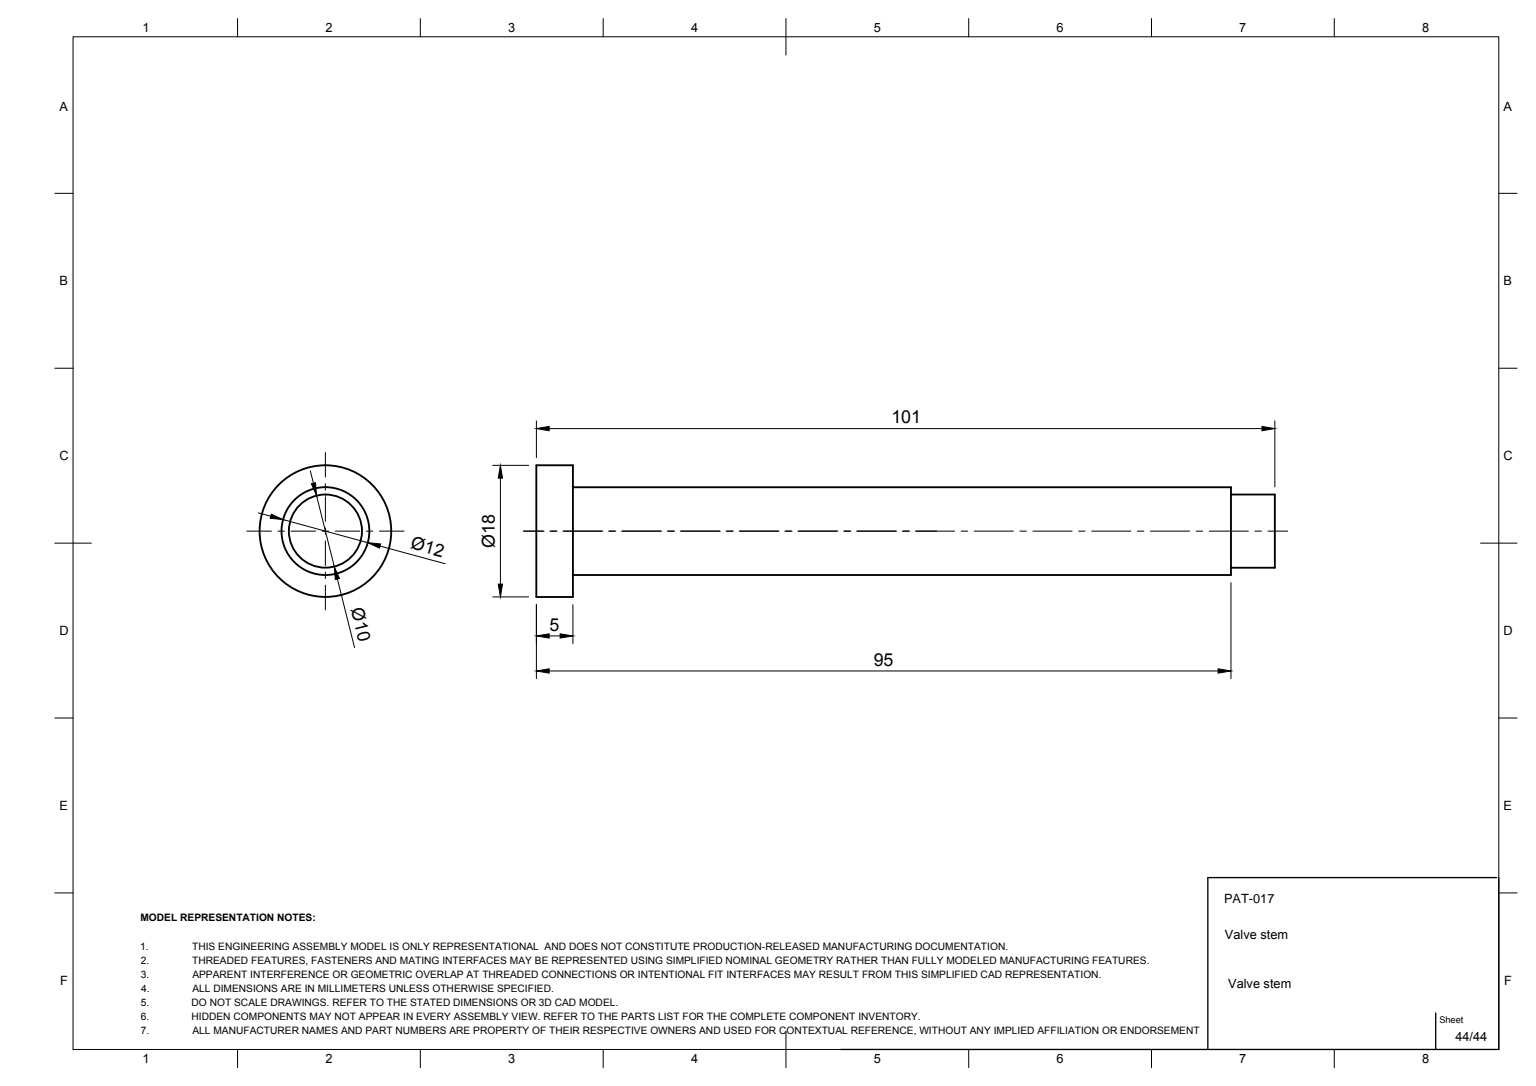
ISO-10303-21;
HEADER;
/* Generated by software containing ST-Developer
 * from STEP Tools, Inc. (www.steptools.com) 
 */

FILE_DESCRIPTION(
/* description */ ('Cam-and-follower valve demonstrator'),
/* implementation_level */ '2;1');

FILE_NAME(
/* name */ 'Valve stem.step',
/* time_stamp */ '2026-10-28T03:25:17-07:00',
/* author */ (''),
/* organization */ (''),
/* preprocessor_version */ 'ST-DEVELOPER v20.2',
/* originating_system */ 'Autodesk Translation Framework v15.17.0.0',
/* authorisation */ '');

FILE_SCHEMA (('AUTOMOTIVE_DESIGN { 1 0 10303 214 3 1 1 }'));
ENDSEC;

DATA;
#10=MECHANICAL_DESIGN_GEOMETRIC_PRESENTATION_REPRESENTATION('',(#453),#12896);
#374=SHAPE_REPRESENTATION_RELATIONSHIP('SRR','None',#13094,#410);
#410=ADVANCED_BREP_SHAPE_REPRESENTATION('',(#493),#12894);
#453=STYLED_ITEM('',(#13344),#493);
#493=MANIFOLD_SOLID_BREP('Body1',#6223);
#655=FACE_BOUND('',#1981,.T.);
#656=FACE_BOUND('',#1988,.T.);
#963=CIRCLE('',#7387,0.9);
#964=CIRCLE('',#7388,0.6);
#965=CIRCLE('',#7390,0.9);
#966=CIRCLE('',#7393,0.5);
#967=CIRCLE('',#7394,0.5);
#968=CIRCLE('',#7397,0.6);
#1090=CYLINDRICAL_SURFACE('',#7389,0.9);
#1091=CYLINDRICAL_SURFACE('',#7392,0.5);
#1092=CYLINDRICAL_SURFACE('',#7396,0.6);
#1452=FACE_OUTER_BOUND('',#1980,.T.);
#1453=FACE_OUTER_BOUND('',#1982,.T.);
#1454=FACE_OUTER_BOUND('',#1983,.T.);
#1455=FACE_OUTER_BOUND('',#1984,.T.);
#1456=FACE_OUTER_BOUND('',#1985,.T.);
#1457=FACE_OUTER_BOUND('',#1986,.T.);
#1458=FACE_OUTER_BOUND('',#1987,.T.);
#1980=EDGE_LOOP('',(#5567));
#1981=EDGE_LOOP('',(#5568));
#1982=EDGE_LOOP('',(#5569,#5570,#5571,#5572));
#1983=EDGE_LOOP('',(#5573));
#1984=EDGE_LOOP('',(#5574,#5575,#5576,#5577));
#1985=EDGE_LOOP('',(#5578));
#1986=EDGE_LOOP('',(#5579,#5580,#5581,#5582));
#1987=EDGE_LOOP('',(#5583));
#1988=EDGE_LOOP('',(#5584));
#2412=LINE('',#12776,#2834);
#2413=LINE('',#12782,#2835);
#2414=LINE('',#12787,#2836);
#2834=VECTOR('',#9369,0.9);
#2835=VECTOR('',#9376,0.5);
#2836=VECTOR('',#9383,0.6);
#3334=VERTEX_POINT('',#12769);
#3335=VERTEX_POINT('',#12771);
#3336=VERTEX_POINT('',#12774);
#3337=VERTEX_POINT('',#12779);
#3338=VERTEX_POINT('',#12781);
#3339=VERTEX_POINT('',#12786);
#4080=EDGE_CURVE('',#3334,#3334,#963,.T.);
#4081=EDGE_CURVE('',#3335,#3335,#964,.T.);
#4082=EDGE_CURVE('',#3336,#3336,#965,.T.);
#4083=EDGE_CURVE('',#3336,#3334,#2412,.T.);
#4084=EDGE_CURVE('',#3337,#3337,#966,.T.);
#4085=EDGE_CURVE('',#3337,#3338,#2413,.T.);
#4086=EDGE_CURVE('',#3338,#3338,#967,.T.);
#4087=EDGE_CURVE('',#3335,#3339,#2414,.T.);
#4088=EDGE_CURVE('',#3339,#3339,#968,.T.);
#5567=ORIENTED_EDGE('',*,*,#4080,.F.);
#5568=ORIENTED_EDGE('',*,*,#4081,.T.);
#5569=ORIENTED_EDGE('',*,*,#4082,.F.);
#5570=ORIENTED_EDGE('',*,*,#4083,.T.);
#5571=ORIENTED_EDGE('',*,*,#4080,.T.);
#5572=ORIENTED_EDGE('',*,*,#4083,.F.);
#5573=ORIENTED_EDGE('',*,*,#4082,.T.);
#5574=ORIENTED_EDGE('',*,*,#4084,.F.);
#5575=ORIENTED_EDGE('',*,*,#4085,.T.);
#5576=ORIENTED_EDGE('',*,*,#4086,.T.);
#5577=ORIENTED_EDGE('',*,*,#4085,.F.);
#5578=ORIENTED_EDGE('',*,*,#4086,.F.);
#5579=ORIENTED_EDGE('',*,*,#4081,.F.);
#5580=ORIENTED_EDGE('',*,*,#4087,.T.);
#5581=ORIENTED_EDGE('',*,*,#4088,.T.);
#5582=ORIENTED_EDGE('',*,*,#4087,.F.);
#5583=ORIENTED_EDGE('',*,*,#4088,.F.);
#5584=ORIENTED_EDGE('',*,*,#4084,.T.);
#5805=PLANE('',#7386);
#5806=PLANE('',#7391);
#5807=PLANE('',#7395);
#5808=PLANE('',#7398);
#6168=ADVANCED_FACE('',(#1452,#655),#5805,.F.);
#6169=ADVANCED_FACE('',(#1453),#1090,.T.);
#6170=ADVANCED_FACE('',(#1454),#5806,.T.);
#6171=ADVANCED_FACE('',(#1455),#1091,.T.);
#6172=ADVANCED_FACE('',(#1456),#5807,.F.);
#6173=ADVANCED_FACE('',(#1457),#1092,.T.);
#6174=ADVANCED_FACE('',(#1458,#656),#5808,.F.);
#6223=CLOSED_SHELL('',(#6168,#6169,#6170,#6171,#6172,#6173,#6174));
#7385=AXIS2_PLACEMENT_3D('',#12767,#9357,#9358);
#7386=AXIS2_PLACEMENT_3D('',#12768,#9359,#9360);
#7387=AXIS2_PLACEMENT_3D('',#12770,#9361,#9362);
#7388=AXIS2_PLACEMENT_3D('',#12772,#9363,#9364);
#7389=AXIS2_PLACEMENT_3D('',#12773,#9365,#9366);
#7390=AXIS2_PLACEMENT_3D('',#12775,#9367,#9368);
#7391=AXIS2_PLACEMENT_3D('',#12777,#9370,#9371);
#7392=AXIS2_PLACEMENT_3D('',#12778,#9372,#9373);
#7393=AXIS2_PLACEMENT_3D('',#12780,#9374,#9375);
#7394=AXIS2_PLACEMENT_3D('',#12783,#9377,#9378);
#7395=AXIS2_PLACEMENT_3D('',#12784,#9379,#9380);
#7396=AXIS2_PLACEMENT_3D('',#12785,#9381,#9382);
#7397=AXIS2_PLACEMENT_3D('',#12788,#9384,#9385);
#7398=AXIS2_PLACEMENT_3D('',#12789,#9386,#9387);
#9357=DIRECTION('axis',(0.,0.,1.));
#9358=DIRECTION('refdir',(1.,0.,0.));
#9359=DIRECTION('center_axis',(0.,0.,1.));
#9360=DIRECTION('ref_axis',(1.,0.,0.));
#9361=DIRECTION('center_axis',(0.,0.,1.));
#9362=DIRECTION('ref_axis',(1.,0.,0.));
#9363=DIRECTION('center_axis',(0.,0.,1.));
#9364=DIRECTION('ref_axis',(1.,0.,0.));
#9365=DIRECTION('center_axis',(0.,0.,1.));
#9366=DIRECTION('ref_axis',(1.,0.,0.));
#9367=DIRECTION('center_axis',(0.,0.,1.));
#9368=DIRECTION('ref_axis',(1.,0.,0.));
#9369=DIRECTION('',(0.,0.,-1.));
#9370=DIRECTION('center_axis',(0.,0.,1.));
#9371=DIRECTION('ref_axis',(1.,0.,0.));
#9372=DIRECTION('center_axis',(0.,0.,1.));
#9373=DIRECTION('ref_axis',(1.,0.,0.));
#9374=DIRECTION('center_axis',(0.,0.,1.));
#9375=DIRECTION('ref_axis',(1.,0.,0.));
#9376=DIRECTION('',(0.,0.,-1.));
#9377=DIRECTION('center_axis',(0.,0.,1.));
#9378=DIRECTION('ref_axis',(1.,0.,0.));
#9379=DIRECTION('center_axis',(0.,0.,1.));
#9380=DIRECTION('ref_axis',(1.,0.,0.));
#9381=DIRECTION('center_axis',(0.,0.,1.));
#9382=DIRECTION('ref_axis',(1.,0.,0.));
#9383=DIRECTION('',(0.,0.,-1.));
#9384=DIRECTION('center_axis',(0.,0.,1.));
#9385=DIRECTION('ref_axis',(1.,0.,0.));
#9386=DIRECTION('center_axis',(0.,0.,1.));
#9387=DIRECTION('ref_axis',(1.,0.,0.));
#12767=CARTESIAN_POINT('',(0.,0.,0.));
#12768=CARTESIAN_POINT('Origin',(0.,0.,16.));
#12769=CARTESIAN_POINT('',(-0.9,-1.10218211923262E-16,16.));
#12770=CARTESIAN_POINT('Origin',(0.,0.,16.));
#12771=CARTESIAN_POINT('',(-0.6,-7.34788079488412E-17,16.));
#12772=CARTESIAN_POINT('Origin',(0.,0.,16.));
#12773=CARTESIAN_POINT('Origin',(0.,0.,16.));
#12774=CARTESIAN_POINT('',(-0.9,-1.10218211923262E-16,16.5));
#12775=CARTESIAN_POINT('Origin',(0.,0.,16.5));
#12776=CARTESIAN_POINT('',(-0.9,-1.10218211923262E-16,16.));
#12777=CARTESIAN_POINT('Origin',(0.,0.,16.5));
#12778=CARTESIAN_POINT('Origin',(0.,0.,6.4));
#12779=CARTESIAN_POINT('',(-0.5,-6.12323399573677E-17,7.));
#12780=CARTESIAN_POINT('Origin',(0.,0.,7.));
#12781=CARTESIAN_POINT('',(-0.5,-6.12323399573677E-17,6.4));
#12782=CARTESIAN_POINT('',(-0.5,-6.12323399573677E-17,6.4));
#12783=CARTESIAN_POINT('Origin',(0.,0.,6.4));
#12784=CARTESIAN_POINT('Origin',(0.,0.,6.4));
#12785=CARTESIAN_POINT('Origin',(0.,0.,7.));
#12786=CARTESIAN_POINT('',(-0.6,-7.34788079488412E-17,7.));
#12787=CARTESIAN_POINT('',(-0.6,-7.34788079488412E-17,7.));
#12788=CARTESIAN_POINT('Origin',(0.,0.,7.));
#12789=CARTESIAN_POINT('Origin',(0.,0.,7.));
#12851=UNCERTAINTY_MEASURE_WITH_UNIT(LENGTH_MEASURE(0.001),#12897,
'DISTANCE_ACCURACY_VALUE',
'Maximum model space distance between geometric entities at asserted c
onnectivities');
#12853=UNCERTAINTY_MEASURE_WITH_UNIT(LENGTH_MEASURE(0.001),#12897,
'DISTANCE_ACCURACY_VALUE',
'Maximum model space distance between geometric entities at asserted c
onnectivities');
#12894=(
GEOMETRIC_REPRESENTATION_CONTEXT(3)
GLOBAL_UNCERTAINTY_ASSIGNED_CONTEXT((#12851))
GLOBAL_UNIT_ASSIGNED_CONTEXT((#12897,#12899,#12900))
REPRESENTATION_CONTEXT('','3D')
);
#12896=(
GEOMETRIC_REPRESENTATION_CONTEXT(3)
GLOBAL_UNCERTAINTY_ASSIGNED_CONTEXT((#12853))
GLOBAL_UNIT_ASSIGNED_CONTEXT((#12897,#12899,#12900))
REPRESENTATION_CONTEXT('','3D')
);
#12897=(
LENGTH_UNIT()
NAMED_UNIT(*)
SI_UNIT(.CENTI.,.METRE.)
);
#12899=(
NAMED_UNIT(*)
PLANE_ANGLE_UNIT()
SI_UNIT($,.RADIAN.)
);
#12900=(
NAMED_UNIT(*)
SI_UNIT($,.STERADIAN.)
SOLID_ANGLE_UNIT()
);
#12941=SHAPE_DEFINITION_REPRESENTATION(#13046,#13094);
#13046=PRODUCT_DEFINITION_SHAPE('',$,#13137);
#13094=SHAPE_REPRESENTATION('',(#7385),#12894);
#13096=PRODUCT_DEFINITION_CONTEXT('part definition',#13224,'design');
#13137=PRODUCT_DEFINITION('Valve stem','Valve stem',#13179,#13096);
#13179=PRODUCT_DEFINITION_FORMATION('',$,#13266);
#13224=APPLICATION_CONTEXT(
'Core Data for Automotive Mechanical Design Process');
#13225=PRODUCT_CONTEXT('part definition',#13224,'mechanical');
#13266=PRODUCT('Valve stem','Valve stem','Valve stem',(#13225));
#13338=COLOUR_RGB('Off White',0.89,0.88,0.83);
#13339=FILL_AREA_STYLE_COLOUR('',#13338);
#13340=FILL_AREA_STYLE('',(#13339));
#13341=SURFACE_STYLE_FILL_AREA(#13340);
#13342=SURFACE_SIDE_STYLE('',(#13341));
#13343=SURFACE_STYLE_USAGE(.BOTH.,#13342);
#13344=PRESENTATION_STYLE_ASSIGNMENT((#13343));
ENDSEC;
END-ISO-10303-21;
